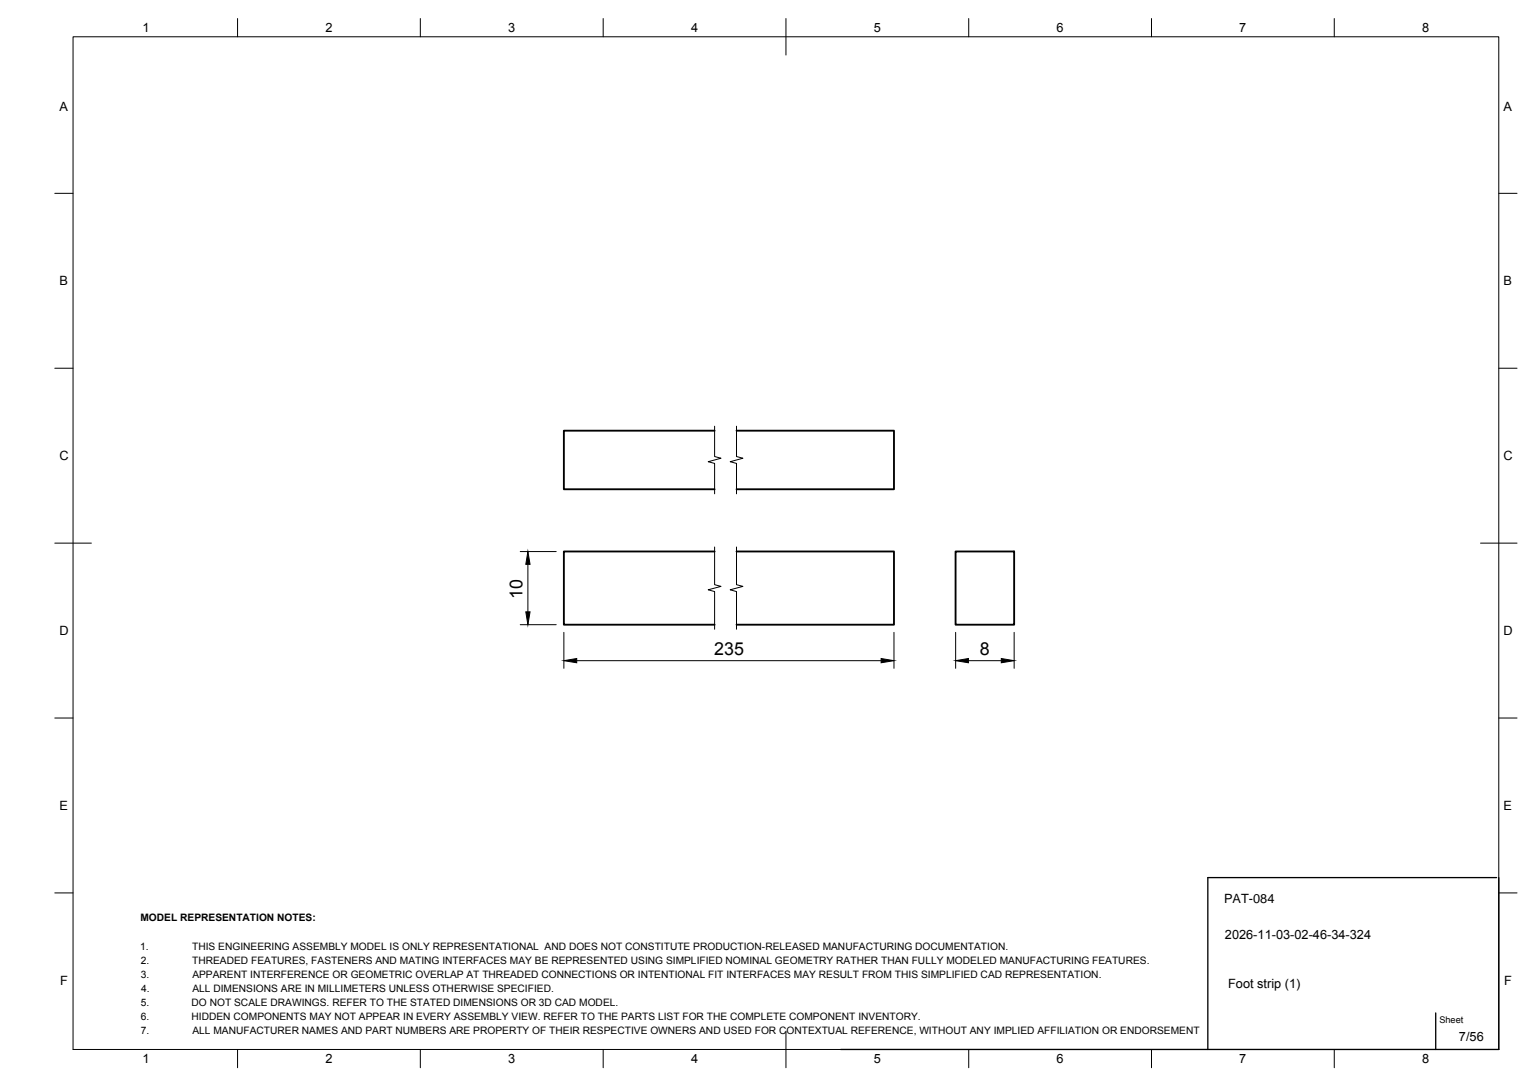
ISO-10303-21;
HEADER;
/* Generated by software containing ST-Developer
 * from STEP Tools, Inc. (www.steptools.com) 
 */

FILE_DESCRIPTION(
/* description */ ('Quick-return (Whitworth) mechanism'),
/* implementation_level */ '2;1');

FILE_NAME(
/* name */ 'Foot strip (1).step',
/* time_stamp */ '2026-10-28T03:25:57-07:00',
/* author */ (''),
/* organization */ (''),
/* preprocessor_version */ 'ST-DEVELOPER v20.2',
/* originating_system */ 'Autodesk Translation Framework v15.17.0.0',
/* authorisation */ '');

FILE_SCHEMA (('AUTOMOTIVE_DESIGN { 1 0 10303 214 3 1 1 }'));
ENDSEC;

DATA;
#10=MECHANICAL_DESIGN_GEOMETRIC_PRESENTATION_REPRESENTATION('',(#492),#14878);
#404=SHAPE_REPRESENTATION_RELATIONSHIP('SRR','None',#15072,#448);
#448=ADVANCED_BREP_SHAPE_REPRESENTATION('',(#544),#14829);
#492=STYLED_ITEM('',(#15392),#544);
#544=MANIFOLD_SOLID_BREP('Body1',#7846);
#794=PLANE('',#8437);
#795=PLANE('',#8438);
#796=PLANE('',#8439);
#797=PLANE('',#8440);
#798=PLANE('',#8441);
#799=PLANE('',#8442);
#1071=FACE_OUTER_BOUND('',#1561,.T.);
#1072=FACE_OUTER_BOUND('',#1562,.T.);
#1073=FACE_OUTER_BOUND('',#1563,.T.);
#1074=FACE_OUTER_BOUND('',#1564,.T.);
#1075=FACE_OUTER_BOUND('',#1565,.T.);
#1076=FACE_OUTER_BOUND('',#1566,.T.);
#1561=EDGE_LOOP('',(#5382,#5383,#5384,#5385));
#1562=EDGE_LOOP('',(#5386,#5387,#5388,#5389));
#1563=EDGE_LOOP('',(#5390,#5391,#5392,#5393));
#1564=EDGE_LOOP('',(#5394,#5395,#5396,#5397));
#1565=EDGE_LOOP('',(#5398,#5399,#5400,#5401));
#1566=EDGE_LOOP('',(#5402,#5403,#5404,#5405));
#2206=LINE('',#12078,#2729);
#2207=LINE('',#12080,#2730);
#2208=LINE('',#12082,#2731);
#2209=LINE('',#12083,#2732);
#2210=LINE('',#12086,#2733);
#2211=LINE('',#12088,#2734);
#2212=LINE('',#12089,#2735);
#2213=LINE('',#12092,#2736);
#2214=LINE('',#12094,#2737);
#2215=LINE('',#12095,#2738);
#2216=LINE('',#12097,#2739);
#2217=LINE('',#12098,#2740);
#2729=VECTOR('',#9541,1.);
#2730=VECTOR('',#9542,1.);
#2731=VECTOR('',#9543,1.);
#2732=VECTOR('',#9544,1.);
#2733=VECTOR('',#9547,1.);
#2734=VECTOR('',#9548,1.);
#2735=VECTOR('',#9549,1.);
#2736=VECTOR('',#9552,1.);
#2737=VECTOR('',#9553,1.);
#2738=VECTOR('',#9554,1.);
#2739=VECTOR('',#9557,1.);
#2740=VECTOR('',#9558,1.);
#3671=VERTEX_POINT('',#12076);
#3672=VERTEX_POINT('',#12077);
#3673=VERTEX_POINT('',#12079);
#3674=VERTEX_POINT('',#12081);
#3675=VERTEX_POINT('',#12085);
#3676=VERTEX_POINT('',#12087);
#3677=VERTEX_POINT('',#12091);
#3678=VERTEX_POINT('',#12093);
#4348=EDGE_CURVE('',#3671,#3672,#2206,.T.);
#4349=EDGE_CURVE('',#3672,#3673,#2207,.T.);
#4350=EDGE_CURVE('',#3674,#3673,#2208,.T.);
#4351=EDGE_CURVE('',#3671,#3674,#2209,.T.);
#4352=EDGE_CURVE('',#3675,#3671,#2210,.T.);
#4353=EDGE_CURVE('',#3676,#3674,#2211,.T.);
#4354=EDGE_CURVE('',#3675,#3676,#2212,.T.);
#4355=EDGE_CURVE('',#3677,#3675,#2213,.T.);
#4356=EDGE_CURVE('',#3678,#3676,#2214,.T.);
#4357=EDGE_CURVE('',#3677,#3678,#2215,.T.);
#4358=EDGE_CURVE('',#3672,#3677,#2216,.T.);
#4359=EDGE_CURVE('',#3673,#3678,#2217,.T.);
#5382=ORIENTED_EDGE('',*,*,#4348,.T.);
#5383=ORIENTED_EDGE('',*,*,#4349,.T.);
#5384=ORIENTED_EDGE('',*,*,#4350,.F.);
#5385=ORIENTED_EDGE('',*,*,#4351,.F.);
#5386=ORIENTED_EDGE('',*,*,#4352,.T.);
#5387=ORIENTED_EDGE('',*,*,#4351,.T.);
#5388=ORIENTED_EDGE('',*,*,#4353,.F.);
#5389=ORIENTED_EDGE('',*,*,#4354,.F.);
#5390=ORIENTED_EDGE('',*,*,#4355,.T.);
#5391=ORIENTED_EDGE('',*,*,#4354,.T.);
#5392=ORIENTED_EDGE('',*,*,#4356,.F.);
#5393=ORIENTED_EDGE('',*,*,#4357,.F.);
#5394=ORIENTED_EDGE('',*,*,#4358,.T.);
#5395=ORIENTED_EDGE('',*,*,#4357,.T.);
#5396=ORIENTED_EDGE('',*,*,#4359,.F.);
#5397=ORIENTED_EDGE('',*,*,#4349,.F.);
#5398=ORIENTED_EDGE('',*,*,#4359,.T.);
#5399=ORIENTED_EDGE('',*,*,#4356,.T.);
#5400=ORIENTED_EDGE('',*,*,#4353,.T.);
#5401=ORIENTED_EDGE('',*,*,#4350,.T.);
#5402=ORIENTED_EDGE('',*,*,#4358,.F.);
#5403=ORIENTED_EDGE('',*,*,#4348,.F.);
#5404=ORIENTED_EDGE('',*,*,#4352,.F.);
#5405=ORIENTED_EDGE('',*,*,#4355,.F.);
#7402=ADVANCED_FACE('',(#1071),#794,.T.);
#7403=ADVANCED_FACE('',(#1072),#795,.T.);
#7404=ADVANCED_FACE('',(#1073),#796,.T.);
#7405=ADVANCED_FACE('',(#1074),#797,.T.);
#7406=ADVANCED_FACE('',(#1075),#798,.T.);
#7407=ADVANCED_FACE('',(#1076),#799,.F.);
#7846=CLOSED_SHELL('',(#7402,#7403,#7404,#7405,#7406,#7407));
#8436=AXIS2_PLACEMENT_3D('',#12074,#9537,#9538);
#8437=AXIS2_PLACEMENT_3D('',#12075,#9539,#9540);
#8438=AXIS2_PLACEMENT_3D('',#12084,#9545,#9546);
#8439=AXIS2_PLACEMENT_3D('',#12090,#9550,#9551);
#8440=AXIS2_PLACEMENT_3D('',#12096,#9555,#9556);
#8441=AXIS2_PLACEMENT_3D('',#12099,#9559,#9560);
#8442=AXIS2_PLACEMENT_3D('',#12100,#9561,#9562);
#9537=DIRECTION('axis',(0.,0.,1.));
#9538=DIRECTION('refdir',(1.,0.,0.));
#9539=DIRECTION('center_axis',(0.,1.,0.));
#9540=DIRECTION('ref_axis',(-1.,0.,0.));
#9541=DIRECTION('',(-1.,0.,0.));
#9542=DIRECTION('',(0.,0.,1.));
#9543=DIRECTION('',(-1.,0.,0.));
#9544=DIRECTION('',(0.,0.,1.));
#9545=DIRECTION('center_axis',(1.,0.,0.));
#9546=DIRECTION('ref_axis',(0.,1.,0.));
#9547=DIRECTION('',(0.,1.,0.));
#9548=DIRECTION('',(0.,1.,0.));
#9549=DIRECTION('',(0.,0.,1.));
#9550=DIRECTION('center_axis',(0.,-1.,0.));
#9551=DIRECTION('ref_axis',(1.,0.,0.));
#9552=DIRECTION('',(1.,0.,0.));
#9553=DIRECTION('',(1.,0.,0.));
#9554=DIRECTION('',(0.,0.,1.));
#9555=DIRECTION('center_axis',(-1.,0.,0.));
#9556=DIRECTION('ref_axis',(0.,-1.,0.));
#9557=DIRECTION('',(0.,-1.,0.));
#9558=DIRECTION('',(0.,-1.,0.));
#9559=DIRECTION('center_axis',(0.,0.,1.));
#9560=DIRECTION('ref_axis',(1.,0.,0.));
#9561=DIRECTION('center_axis',(0.,0.,1.));
#9562=DIRECTION('ref_axis',(1.,0.,0.));
#12074=CARTESIAN_POINT('',(0.,0.,0.));
#12075=CARTESIAN_POINT('Origin',(21.,20.,-0.8));
#12076=CARTESIAN_POINT('',(21.,20.,-0.8));
#12077=CARTESIAN_POINT('',(20.,20.,-0.8));
#12078=CARTESIAN_POINT('',(21.,20.,-0.8));
#12079=CARTESIAN_POINT('',(20.,20.,0.));
#12080=CARTESIAN_POINT('',(20.,20.,-0.8));
#12081=CARTESIAN_POINT('',(21.,20.,0.));
#12082=CARTESIAN_POINT('',(21.,20.,0.));
#12083=CARTESIAN_POINT('',(21.,20.,-0.8));
#12084=CARTESIAN_POINT('Origin',(21.,-3.5,-0.8));
#12085=CARTESIAN_POINT('',(21.,-3.5,-0.8));
#12086=CARTESIAN_POINT('',(21.,-3.5,-0.8));
#12087=CARTESIAN_POINT('',(21.,-3.5,0.));
#12088=CARTESIAN_POINT('',(21.,-3.5,0.));
#12089=CARTESIAN_POINT('',(21.,-3.5,-0.8));
#12090=CARTESIAN_POINT('Origin',(20.,-3.5,-0.8));
#12091=CARTESIAN_POINT('',(20.,-3.5,-0.8));
#12092=CARTESIAN_POINT('',(20.,-3.5,-0.8));
#12093=CARTESIAN_POINT('',(20.,-3.5,0.));
#12094=CARTESIAN_POINT('',(20.,-3.5,0.));
#12095=CARTESIAN_POINT('',(20.,-3.5,-0.8));
#12096=CARTESIAN_POINT('Origin',(20.,20.,-0.8));
#12097=CARTESIAN_POINT('',(20.,20.,-0.8));
#12098=CARTESIAN_POINT('',(20.,20.,0.));
#12099=CARTESIAN_POINT('Origin',(20.5,8.25,0.));
#12100=CARTESIAN_POINT('Origin',(20.5,8.25,-0.8));
#14775=UNCERTAINTY_MEASURE_WITH_UNIT(LENGTH_MEASURE(0.001),#14879,
'DISTANCE_ACCURACY_VALUE',
'Maximum model space distance between geometric entities at asserted c
onnectivities');
#14824=UNCERTAINTY_MEASURE_WITH_UNIT(LENGTH_MEASURE(0.001),#14879,
'DISTANCE_ACCURACY_VALUE',
'Maximum model space distance between geometric entities at asserted c
onnectivities');
#14829=(
GEOMETRIC_REPRESENTATION_CONTEXT(3)
GLOBAL_UNCERTAINTY_ASSIGNED_CONTEXT((#14775))
GLOBAL_UNIT_ASSIGNED_CONTEXT((#14879,#14881,#14882))
REPRESENTATION_CONTEXT('','3D')
);
#14878=(
GEOMETRIC_REPRESENTATION_CONTEXT(3)
GLOBAL_UNCERTAINTY_ASSIGNED_CONTEXT((#14824))
GLOBAL_UNIT_ASSIGNED_CONTEXT((#14879,#14881,#14882))
REPRESENTATION_CONTEXT('','3D')
);
#14879=(
LENGTH_UNIT()
NAMED_UNIT(*)
SI_UNIT(.CENTI.,.METRE.)
);
#14881=(
NAMED_UNIT(*)
PLANE_ANGLE_UNIT()
SI_UNIT($,.RADIAN.)
);
#14882=(
NAMED_UNIT(*)
SI_UNIT($,.STERADIAN.)
SOLID_ANGLE_UNIT()
);
#14887=SHAPE_DEFINITION_REPRESENTATION(#14940,#15072);
#14940=PRODUCT_DEFINITION_SHAPE('',$,#15126);
#15072=SHAPE_REPRESENTATION('',(#8436),#14829);
#15121=PRODUCT_DEFINITION_CONTEXT('part definition',#15282,'design');
#15126=PRODUCT_DEFINITION('Foot strip (1)','Foot strip (1)',#15179,#15121);
#15179=PRODUCT_DEFINITION_FORMATION('',$,#15288);
#15282=APPLICATION_CONTEXT(
'Core Data for Automotive Mechanical Design Process');
#15283=PRODUCT_CONTEXT('part definition',#15282,'mechanical');
#15288=PRODUCT('Foot strip (1)','Foot strip (1)','Foot strip (1)',(#15283));
#15386=COLOUR_RGB('Light Blue',0.38,0.62,0.78);
#15387=FILL_AREA_STYLE_COLOUR('',#15386);
#15388=FILL_AREA_STYLE('',(#15387));
#15389=SURFACE_STYLE_FILL_AREA(#15388);
#15390=SURFACE_SIDE_STYLE('',(#15389));
#15391=SURFACE_STYLE_USAGE(.BOTH.,#15390);
#15392=PRESENTATION_STYLE_ASSIGNMENT((#15391));
ENDSEC;
END-ISO-10303-21;
